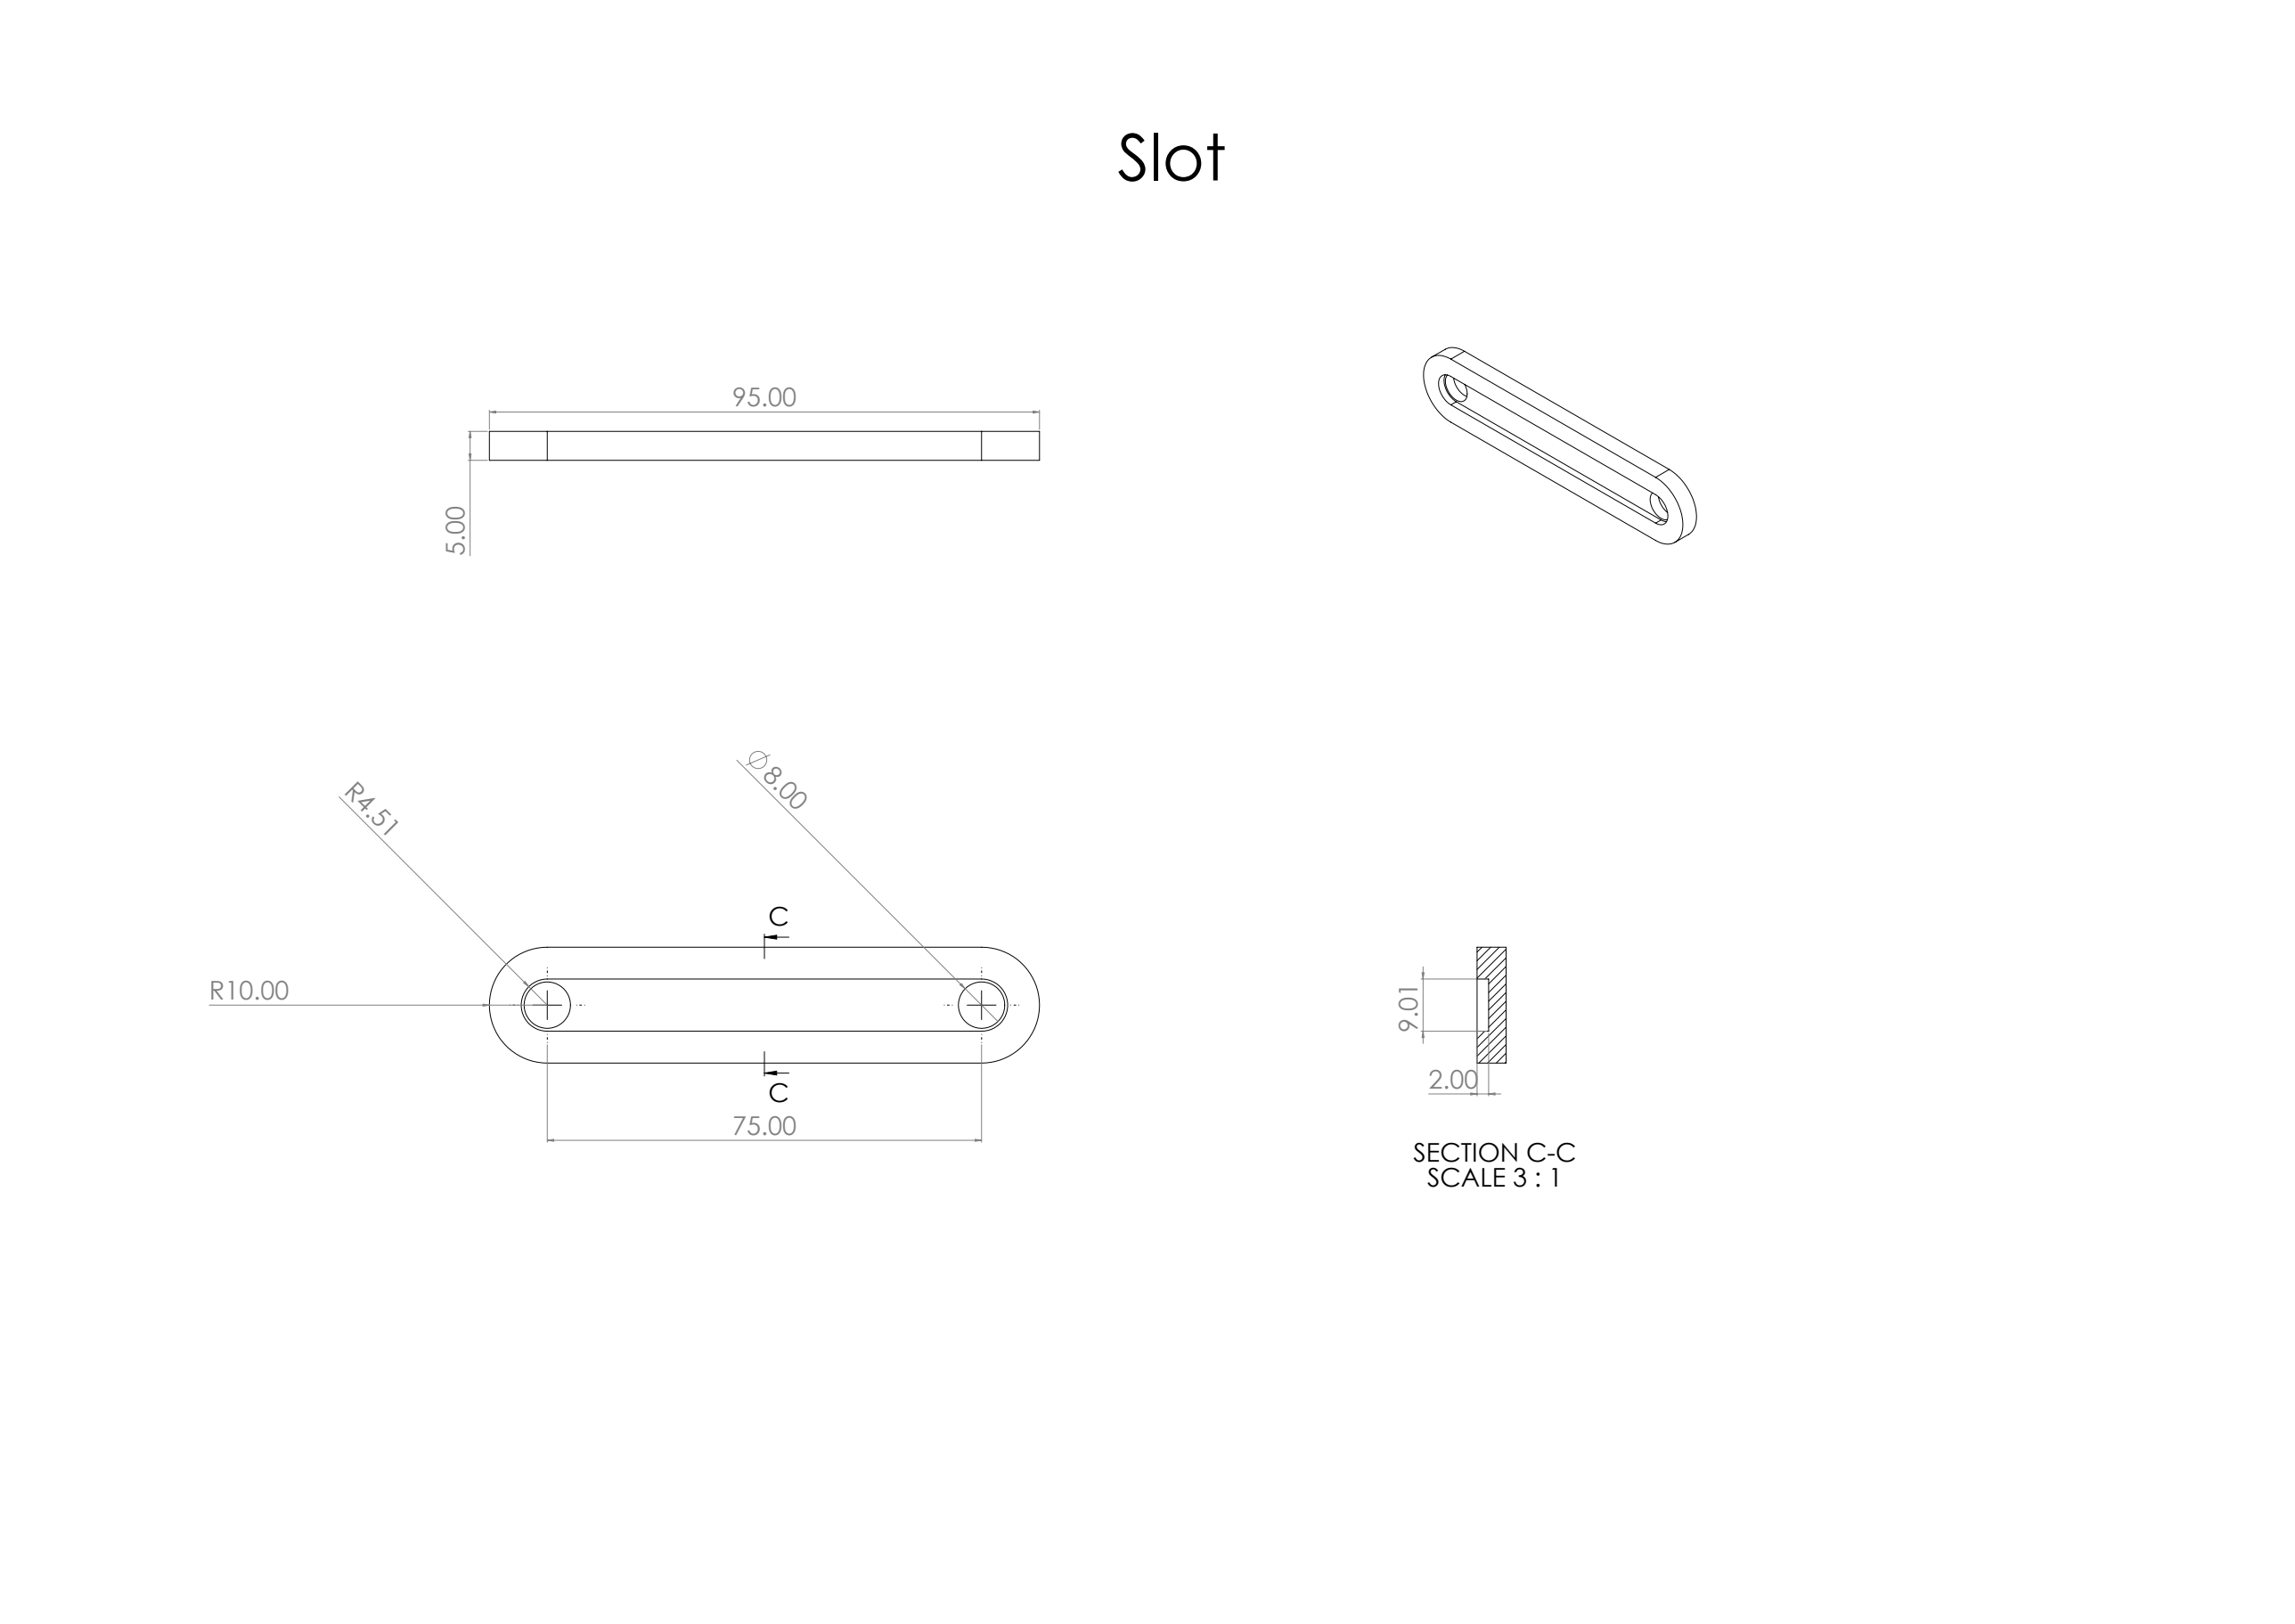
ISO-10303-21;
HEADER;
FILE_DESCRIPTION (('STEP AP214'),
    '1' );
FILE_NAME ('Slot.step',
    '2026-10-24T21:31:31',
    ( '' ),
    ( '' ),
    'SwSTEP 2.0',
    'SolidWorks 2025',
    '' );
FILE_SCHEMA (( 'AUTOMOTIVE_DESIGN' ));
ENDSEC;

DATA;
#16=CARTESIAN_POINT ( 'NONE',  ( 58.00000000000000711, -2.249290599286311032, 36.00000000000012079 ) ) ;
#145=ORIENTED_EDGE ( 'NONE', *, *, #4688, .T. ) ;
#181=CIRCLE ( 'NONE', #13427, 4.505436745857433145 ) ;
#184=ORIENTED_EDGE ( 'NONE', *, *, #4181, .F. ) ;
#194=CARTESIAN_POINT ( 'NONE',  ( -16.99999999999998579, -2.249290599286303927, 33.00000000000012790 ) ) ;
#251=VERTEX_POINT ( 'NONE', #11733 ) ;
#262=ADVANCED_FACE ( 'NONE', ( #2849 ), #1628, .F. ) ;
#272=FACE_OUTER_BOUND ( 'NONE', #12686, .T. ) ;
#287=CIRCLE ( 'NONE', #2244, 4.000000000000000000 ) ;
#323=CARTESIAN_POINT ( 'NONE',  ( -16.99999999999998579, -2.249290599286303927, 38.00000000000012079 ) ) ;
#328=CARTESIAN_POINT ( 'NONE',  ( 62.50543674585744469, -2.249290599286311032, 36.00000000000012079 ) ) ;
#339=EDGE_CURVE ( 'NONE', #4676, #369, #5590, .T. ) ;
#357=ORIENTED_EDGE ( 'NONE', *, *, #11069, .T. ) ;
#369=VERTEX_POINT ( 'NONE', #6019 ) ;
#394=DIRECTION ( 'NONE',  ( 1.000000000000000000, -9.251858538542971581E-17, 0.000000000000000000 ) ) ;
#405=CARTESIAN_POINT ( 'NONE',  ( -16.99999999999998579, -12.24929059928630437, 38.00000000000012079 ) ) ;
#428=DIRECTION ( 'NONE',  ( 0.000000000000000000, 0.000000000000000000, 1.000000000000000000 ) ) ;
#442=DIRECTION ( 'NONE',  ( 0.000000000000000000, 0.000000000000000000, 1.000000000000000000 ) ) ;
#472=LINE ( 'NONE', #13474, #12021 ) ;
#510=DIRECTION ( 'NONE',  ( 1.000000000000000000, 0.000000000000000000, 0.000000000000000000 ) ) ;
#513=VECTOR ( 'NONE', #15204, 1000.000000000000000 ) ;
#530=AXIS2_PLACEMENT_3D ( 'NONE', #3937, #5033, #8635 ) ;
#543=CARTESIAN_POINT ( 'NONE',  ( -16.99999999999998579, -2.249290599286303927, 38.00000000000012079 ) ) ;
#557=CARTESIAN_POINT ( 'NONE',  ( -16.99999999999998579, 2.256146146571129218, 38.00000000000012079 ) ) ;
#771=CARTESIAN_POINT ( 'NONE',  ( -20.99999999999998579, -2.249290599286303927, 38.00000000000012079 ) ) ;
#810=LINE ( 'NONE', #13901, #15019 ) ;
#898=DIRECTION ( 'NONE',  ( 1.000000000000000000, 0.000000000000000000, 0.000000000000000000 ) ) ;
#902=EDGE_CURVE ( 'NONE', #251, #11798, #9174, .T. ) ;
#905=PRODUCT_DEFINITION ( 'UNKNOWN', '', #1171, #3354 ) ;
#907=CARTESIAN_POINT ( 'NONE',  ( -26.99999999999998934, -2.249290599286303927, 38.00000000000012079 ) ) ;
#963=CARTESIAN_POINT ( 'NONE',  ( 62.00000000000001421, -2.249290599286310588, 33.00000000000012790 ) ) ;
#966=LINE ( 'NONE', #2988, #12194 ) ;
#976=ORIENTED_EDGE ( 'NONE', *, *, #9709, .T. ) ;
#1001=DIRECTION ( 'NONE',  ( 1.000000000000000000, 0.000000000000000000, 0.000000000000000000 ) ) ;
#1011=CARTESIAN_POINT ( 'NONE',  ( -12.99999999999998757, -2.249290599286303483, 36.00000000000012079 ) ) ;
#1066=ORIENTED_EDGE ( 'NONE', *, *, #11069, .F. ) ;
#1085=DIRECTION ( 'NONE',  ( -0.000000000000000000, -0.000000000000000000, -1.000000000000000000 ) ) ;
#1098=FACE_OUTER_BOUND ( 'NONE', #13950, .T. ) ;
#1114=CARTESIAN_POINT ( 'NONE',  ( -16.99999999999998579, -2.249290599286303927, 36.00000000000012079 ) ) ;
#1139=EDGE_CURVE ( 'NONE', #4676, #7142, #8068, .T. ) ;
#1149=ORIENTED_EDGE ( 'NONE', *, *, #11411, .F. ) ;
#1171=PRODUCT_DEFINITION_FORMATION_WITH_SPECIFIED_SOURCE ( 'ANY', '', #1909, .NOT_KNOWN. ) ;
#1196=DIRECTION ( 'NONE',  ( -0.000000000000000000, -0.000000000000000000, 1.000000000000000000 ) ) ;
#1206=ORIENTED_EDGE ( 'NONE', *, *, #9236, .T. ) ;
#1226=EDGE_CURVE ( 'NONE', #5867, #10383, #2818, .T. ) ;
#1241=EDGE_LOOP ( 'NONE', ( #9052, #8384, #14542, #4784 ) ) ;
#1272=VECTOR ( 'NONE', #1085, 1000.000000000000000 ) ;
#1276=AXIS2_PLACEMENT_3D ( 'NONE', #9205, #12823, #13888 ) ;
#1299=VECTOR ( 'NONE', #2746, 1000.000000000000000 ) ;
#1360=CYLINDRICAL_SURFACE ( 'NONE', #11358, 10.00000000000000178 ) ;
#1372=ORIENTED_EDGE ( 'NONE', *, *, #3914, .F. ) ;
#1415=AXIS2_PLACEMENT_3D ( 'NONE', #1771, #6471, #12394 ) ;
#1418=CARTESIAN_POINT ( 'NONE',  ( -16.99999999999998579, -6.754727345143736628, 36.00000000000012079 ) ) ;
#1429=EDGE_LOOP ( 'NONE', ( #13416, #7963, #11470, #145 ) ) ;
#1432=ADVANCED_FACE ( 'NONE', ( #12427 ), #1879, .F. ) ;
#1435=ORIENTED_EDGE ( 'NONE', *, *, #5988, .T. ) ;
#1499=DIRECTION ( 'NONE',  ( 0.000000000000000000, 0.000000000000000000, 1.000000000000000000 ) ) ;
#1548=ADVANCED_FACE ( 'NONE', ( #8125 ), #12828, .F. ) ;
#1573=AXIS2_PLACEMENT_3D ( 'NONE', #13753, #7834, #7985 ) ;
#1575=CARTESIAN_POINT ( 'NONE',  ( 58.00000000000000711, -12.24929059928630970, 33.00000000000012790 ) ) ;
#1602=ORIENTED_EDGE ( 'NONE', *, *, #13204, .F. ) ;
#1609=EDGE_LOOP ( 'NONE', ( #11446, #15210 ) ) ;
#1611=EDGE_CURVE ( 'NONE', #11349, #2219, #7955, .T. ) ;
#1628=CYLINDRICAL_SURFACE ( 'NONE', #13220, 4.505436745857433145 ) ;
#1673=DIRECTION ( 'NONE',  ( 1.000000000000000000, 0.000000000000000000, -0.000000000000000000 ) ) ;
#1699=CARTESIAN_POINT ( 'NONE',  ( 58.00000000000000711, -2.249290599286311032, 36.00000000000012079 ) ) ;
#1700=ADVANCED_BREP_SHAPE_REPRESENTATION ( '', ( #9466, #6315 ), #11962 ) ;
#1717=LINE ( 'NONE', #8951, #3460 ) ;
#1771=CARTESIAN_POINT ( 'NONE',  ( 58.00000000000000711, -2.249290599286311032, 36.00000000000012079 ) ) ;
#1776=DIRECTION ( 'NONE',  ( 0.000000000000000000, 0.000000000000000000, 1.000000000000000000 ) ) ;
#1804=FACE_BOUND ( 'NONE', #3358, .T. ) ;
#1835=DIRECTION ( 'NONE',  ( -0.000000000000000000, -0.000000000000000000, -1.000000000000000000 ) ) ;
#1842=FACE_OUTER_BOUND ( 'NONE', #5321, .T. ) ;
#1845=CARTESIAN_POINT ( 'NONE',  ( 58.00000000000000711, 2.256146146571122113, 38.00000000000012079 ) ) ;
#1853=( NAMED_UNIT ( * ) PLANE_ANGLE_UNIT ( ) SI_UNIT ( $, .RADIAN. ) );
#1879=PLANE ( 'NONE',  #6472 ) ;
#1890=DIRECTION ( 'NONE',  ( 0.000000000000000000, 0.000000000000000000, 1.000000000000000000 ) ) ;
#1898=AXIS2_PLACEMENT_3D ( 'NONE', #12311, #6466, #14548 ) ;
#1904=AXIS2_PLACEMENT_3D ( 'NONE', #3072, #1835, #7844 ) ;
#1906=FACE_OUTER_BOUND ( 'NONE', #7243, .T. ) ;
#1909=PRODUCT ( 'Slot', 'Slot', '', ( #13321 ) ) ;
#1955=FACE_OUTER_BOUND ( 'NONE', #5403, .T. ) ;
#1975=CARTESIAN_POINT ( 'NONE',  ( -16.99999999999998579, -2.249290599286303927, 36.00000000000012079 ) ) ;
#2020=VECTOR ( 'NONE', #2381, 1000.000000000000000 ) ;
#2025=PLANE ( 'NONE',  #9342 ) ;
#2033=AXIS2_PLACEMENT_3D ( 'NONE', #3160, #1776, #10090 ) ;
#2040=CYLINDRICAL_SURFACE ( 'NONE', #3467, 10.00000000000000178 ) ;
#2068=LINE ( 'NONE', #4686, #10105 ) ;
#2132=CIRCLE ( 'NONE', #8294, 4.000000000000000000 ) ;
#2198=DIRECTION ( 'NONE',  ( 1.000000000000000000, 0.000000000000000000, 0.000000000000000000 ) ) ;
#2219=VERTEX_POINT ( 'NONE', #1845 ) ;
#2240=ORIENTED_EDGE ( 'NONE', *, *, #1611, .F. ) ;
#2244=AXIS2_PLACEMENT_3D ( 'NONE', #3620, #8329, #6091 ) ;
#2296=DIRECTION ( 'NONE',  ( 1.000000000000000000, 0.000000000000000000, 0.000000000000000000 ) ) ;
#2306=AXIS2_PLACEMENT_3D ( 'NONE', #4421, #12665, #2198 ) ;
#2323=EDGE_CURVE ( 'NONE', #369, #4676, #10110, .T. ) ;
#2381=DIRECTION ( 'NONE',  ( -1.000000000000000000, 2.312964634635742895E-17, -0.000000000000000000 ) ) ;
#2399=FACE_OUTER_BOUND ( 'NONE', #1241, .T. ) ;
#2462=LINE ( 'NONE', #7151, #2020 ) ;
#2521=EDGE_CURVE ( 'NONE', #4675, #11128, #287, .T. ) ;
#2523=AXIS2_PLACEMENT_3D ( 'NONE', #323, #6178, #9568 ) ;
#2530=EDGE_LOOP ( 'NONE', ( #5795, #11208, #11838, #4778 ) ) ;
#2604=ORIENTED_EDGE ( 'NONE', *, *, #9709, .F. ) ;
#2676=ORIENTED_EDGE ( 'NONE', *, *, #3302, .F. ) ;
#2701=AXIS2_PLACEMENT_3D ( 'NONE', #12923, #7426, #2296 ) ;
#2709=ADVANCED_FACE ( 'NONE', ( #1955 ), #2040, .T. ) ;
#2737=ORIENTED_EDGE ( 'NONE', *, *, #5225, .T. ) ;
#2746=DIRECTION ( 'NONE',  ( -1.000000000000000000, 2.312964634635742895E-17, -0.000000000000000000 ) ) ;
#2749=CARTESIAN_POINT ( 'NONE',  ( 58.00000000000000711, -2.249290599286311032, 36.00000000000012079 ) ) ;
#2762=AXIS2_PLACEMENT_3D ( 'NONE', #16, #11860, #1001 ) ;
#2789=DIRECTION ( 'NONE',  ( -0.000000000000000000, -0.000000000000000000, -1.000000000000000000 ) ) ;
#2818=LINE ( 'NONE', #10981, #1299 ) ;
#2829=CARTESIAN_POINT ( 'NONE',  ( 58.00000000000000711, 2.256146146571122113, 36.00000000000012079 ) ) ;
#2838=ORIENTED_EDGE ( 'NONE', *, *, #13570, .T. ) ;
#2849=FACE_OUTER_BOUND ( 'NONE', #9522, .T. ) ;
#2877=CARTESIAN_POINT ( 'NONE',  ( 58.00000000000000711, 7.750709400713694741, 33.00000000000012790 ) ) ;
#2924=EDGE_CURVE ( 'NONE', #10383, #8896, #5822, .T. ) ;
#2931=CARTESIAN_POINT ( 'NONE',  ( -16.99999999999998579, 2.256146146571129218, 36.00000000000012079 ) ) ;
#2939=CARTESIAN_POINT ( 'NONE',  ( 54.00000000000000711, -2.249290599286311032, 33.00000000000012790 ) ) ;
#2968=EDGE_CURVE ( 'NONE', #6172, #4927, #4433, .T. ) ;
#2976=CARTESIAN_POINT ( 'NONE',  ( -16.99999999999998579, -2.249290599286303927, 38.00000000000012079 ) ) ;
#2980=VECTOR ( 'NONE', #14639, 1000.000000000000000 ) ;
#2988=CARTESIAN_POINT ( 'NONE',  ( 58.00000000000000711, -6.754727345143743733, 36.00000000000012079 ) ) ;
#2991=AXIS2_PLACEMENT_3D ( 'NONE', #10271, #4410, #5656 ) ;
#3024=ORIENTED_EDGE ( 'NONE', *, *, #8643, .T. ) ;
#3060=CARTESIAN_POINT ( 'NONE',  ( 58.00000000000000711, -2.249290599286311032, 38.00000000000012079 ) ) ;
#3072=CARTESIAN_POINT ( 'NONE',  ( -16.99999999999998579, -2.249290599286303927, 38.00000000000012079 ) ) ;
#3114=SHAPE_REPRESENTATION ( 'Slot', ( #6315 ), #11962 ) ;
#3124=ORIENTED_EDGE ( 'NONE', *, *, #3628, .F. ) ;
#3160=CARTESIAN_POINT ( 'NONE',  ( 58.00000000000000711, -2.249290599286311032, 33.00000000000012790 ) ) ;
#3197=AXIS2_PLACEMENT_3D ( 'NONE', #11203, #13594, #5213 ) ;
#3206=DIRECTION ( 'NONE',  ( 1.000000000000000000, 0.000000000000000000, 0.000000000000000000 ) ) ;
#3220=APPLICATION_CONTEXT ( 'automotive_design' ) ;
#3302=EDGE_CURVE ( 'NONE', #369, #13514, #472, .T. ) ;
#3310=EDGE_CURVE ( 'NONE', #5867, #13804, #7330, .T. ) ;
#3329=CARTESIAN_POINT ( 'NONE',  ( 58.00000000000000711, 2.256146146571122113, 36.00000000000012079 ) ) ;
#3333=VERTEX_POINT ( 'NONE', #10952 ) ;
#3354=PRODUCT_DEFINITION_CONTEXT ( 'detailed design', #8324, 'design' ) ;
#3358=EDGE_LOOP ( 'NONE', ( #10086, #3124 ) ) ;
#3416=DIRECTION ( 'NONE',  ( 1.000000000000000000, -2.312964634635742895E-17, 0.000000000000000000 ) ) ;
#3451=EDGE_LOOP ( 'NONE', ( #2676, #5349, #13902, #11604 ) ) ;
#3460=VECTOR ( 'NONE', #13640, 1000.000000000000000 ) ;
#3467=AXIS2_PLACEMENT_3D ( 'NONE', #7974, #4263, #13660 ) ;
#3516=DIRECTION ( 'NONE',  ( 1.000000000000000000, 0.000000000000000000, 0.000000000000000000 ) ) ;
#3535=ORIENTED_EDGE ( 'NONE', *, *, #14400, .T. ) ;
#3583=ADVANCED_FACE ( 'NONE', ( #10554 ), #7862, .F. ) ;
#3620=CARTESIAN_POINT ( 'NONE',  ( -16.99999999999998579, -2.249290599286303927, 33.00000000000012790 ) ) ;
#3628=EDGE_CURVE ( 'NONE', #11798, #251, #12783, .T. ) ;
#3732=EDGE_LOOP ( 'NONE', ( #9194, #12086, #1206, #5379, #12814 ) ) ;
#3799=EDGE_CURVE ( 'NONE', #13514, #7142, #9341, .T. ) ;
#3900=ORIENTED_EDGE ( 'NONE', *, *, #6796, .F. ) ;
#3914=EDGE_CURVE ( 'NONE', #13135, #5290, #9962, .T. ) ;
#3930=DIRECTION ( 'NONE',  ( -1.000000000000000000, 9.251858538542971581E-17, 0.000000000000000000 ) ) ;
#3937=CARTESIAN_POINT ( 'NONE',  ( -16.99999999999998579, -2.249290599286303927, 38.00000000000012079 ) ) ;
#3949=ORIENTED_EDGE ( 'NONE', *, *, #3914, .T. ) ;
#3965=CIRCLE ( 'NONE', #530, 10.00000000000000000 ) ;
#4005=DIRECTION ( 'NONE',  ( -0.000000000000000000, -0.000000000000000000, -1.000000000000000000 ) ) ;
#4044=CYLINDRICAL_SURFACE ( 'NONE', #3197, 10.00000000000000178 ) ;
#4082=CARTESIAN_POINT ( 'NONE',  ( 0.000000000000000000, 0.000000000000000000, 0.000000000000000000 ) ) ;
#4105=FACE_BOUND ( 'NONE', #10933, .T. ) ;
#4135=DIRECTION ( 'NONE',  ( 0.000000000000000000, 0.000000000000000000, 1.000000000000000000 ) ) ;
#4175=FACE_BOUND ( 'NONE', #1609, .T. ) ;
#4181=EDGE_CURVE ( 'NONE', #4272, #13804, #6672, .T. ) ;
#4189=PLANE ( 'NONE',  #8535 ) ;
#4223=DIRECTION ( 'NONE',  ( 9.251858538542971581E-17, 1.000000000000000000, 0.000000000000000000 ) ) ;
#4263=DIRECTION ( 'NONE',  ( -0.000000000000000000, -0.000000000000000000, -1.000000000000000000 ) ) ;
#4272=VERTEX_POINT ( 'NONE', #1575 ) ;
#4288=CYLINDRICAL_SURFACE ( 'NONE', #1904, 4.000000000000000000 ) ;
#4314=ORIENTED_EDGE ( 'NONE', *, *, #7498, .T. ) ;
#4317=ADVANCED_FACE ( 'NONE', ( #272 ), #11955, .F. ) ;
#4357=LINE ( 'NONE', #11275, #11956 ) ;
#4410=DIRECTION ( 'NONE',  ( 0.000000000000000000, 0.000000000000000000, 1.000000000000000000 ) ) ;
#4421=CARTESIAN_POINT ( 'NONE',  ( -16.99999999999998579, -2.249290599286303927, 36.00000000000012079 ) ) ;
#4433=CIRCLE ( 'NONE', #12304, 4.505436745857433145 ) ;
#4512=VERTEX_POINT ( 'NONE', #14010 ) ;
#4525=DIRECTION ( 'NONE',  ( -0.000000000000000000, -0.000000000000000000, -1.000000000000000000 ) ) ;
#4563=CARTESIAN_POINT ( 'NONE',  ( -16.99999999999998579, -12.24929059928630437, 38.00000000000012079 ) ) ;
#4656=VECTOR ( 'NONE', #2789, 1000.000000000000000 ) ;
#4666=AXIS2_PLACEMENT_3D ( 'NONE', #15168, #10475, #8009 ) ;
#4675=VERTEX_POINT ( 'NONE', #11547 ) ;
#4676=VERTEX_POINT ( 'NONE', #13948 ) ;
#4686=CARTESIAN_POINT ( 'NONE',  ( 62.50543674585744469, -2.249290599286311032, 36.00000000000012079 ) ) ;
#4688=EDGE_CURVE ( 'NONE', #14170, #9032, #11314, .T. ) ;
#4751=DIRECTION ( 'NONE',  ( 1.000000000000000000, 0.000000000000000000, 0.000000000000000000 ) ) ;
#4778=ORIENTED_EDGE ( 'NONE', *, *, #9015, .T. ) ;
#4784=ORIENTED_EDGE ( 'NONE', *, *, #11562, .T. ) ;
#4893=EDGE_LOOP ( 'NONE', ( #1372, #8177, #14989, #976 ) ) ;
#4898=DIRECTION ( 'NONE',  ( 0.000000000000000000, 0.000000000000000000, 1.000000000000000000 ) ) ;
#4916=CARTESIAN_POINT ( 'NONE',  ( -16.99999999999998579, 2.256146146571129218, 36.00000000000012079 ) ) ;
#4922=ORIENTED_EDGE ( 'NONE', *, *, #13204, .T. ) ;
#4923=EDGE_CURVE ( 'NONE', #4512, #6172, #14408, .T. ) ;
#4927=VERTEX_POINT ( 'NONE', #328 ) ;
#4962=DIRECTION ( 'NONE',  ( 1.000000000000000000, -9.251858538542971581E-17, 0.000000000000000000 ) ) ;
#5033=DIRECTION ( 'NONE',  ( 0.000000000000000000, 0.000000000000000000, 1.000000000000000000 ) ) ;
#5093=LINE ( 'NONE', #13389, #8004 ) ;
#5097=DIRECTION ( 'NONE',  ( 1.000000000000000000, 0.000000000000000000, 0.000000000000000000 ) ) ;
#5163=CARTESIAN_POINT ( 'NONE',  ( 58.00000000000000711, -6.754727345143743733, 38.00000000000012079 ) ) ;
#5182=CIRCLE ( 'NONE', #11818, 4.505436745857433145 ) ;
#5213=DIRECTION ( 'NONE',  ( -1.000000000000000000, 0.000000000000000000, 0.000000000000000000 ) ) ;
#5225=EDGE_CURVE ( 'NONE', #13804, #8896, #2462, .T. ) ;
#5242=PLANE ( 'NONE',  #8272 ) ;
#5290=VERTEX_POINT ( 'NONE', #8679 ) ;
#5321=EDGE_LOOP ( 'NONE', ( #10858, #9774, #1602, #5841 ) ) ;
#5349=ORIENTED_EDGE ( 'NONE', *, *, #2323, .T. ) ;
#5362=DIRECTION ( 'NONE',  ( 0.000000000000000000, 0.000000000000000000, 1.000000000000000000 ) ) ;
#5379=ORIENTED_EDGE ( 'NONE', *, *, #8061, .T. ) ;
#5403=EDGE_LOOP ( 'NONE', ( #11144, #3949, #357, #6231 ) ) ;
#5432=DIRECTION ( 'NONE',  ( -1.000000000000000000, 6.938893903907228378E-17, 0.000000000000000000 ) ) ;
#5471=ADVANCED_FACE ( 'NONE', ( #14671 ), #10296, .F. ) ;
#5494=AXIS2_PLACEMENT_3D ( 'NONE', #1975, #4135, #898 ) ;
#5561=DIRECTION ( 'NONE',  ( -0.000000000000000000, -0.000000000000000000, -1.000000000000000000 ) ) ;
#5578=ORIENTED_EDGE ( 'NONE', *, *, #2968, .T. ) ;
#5590=CIRCLE ( 'NONE', #1415, 4.000000000000003553 ) ;
#5648=( GEOMETRIC_REPRESENTATION_CONTEXT ( 3 ) GLOBAL_UNCERTAINTY_ASSIGNED_CONTEXT ( ( #13207 ) ) GLOBAL_UNIT_ASSIGNED_CONTEXT ( ( #6778, #1853, #9097 ) ) REPRESENTATION_CONTEXT ( 'NONE', 'WORKASPACE' ) );
#5656=DIRECTION ( 'NONE',  ( 1.000000000000000000, 0.000000000000000000, -0.000000000000000000 ) ) ;
#5688=AXIS2_PLACEMENT_3D ( 'NONE', #10989, #5362, #510 ) ;
#5760=CARTESIAN_POINT ( 'NONE',  ( -16.99999999999998579, 2.256146146571129218, 38.00000000000012079 ) ) ;
#5793=ADVANCED_FACE ( 'NONE', ( #9904 ), #1360, .T. ) ;
#5795=ORIENTED_EDGE ( 'NONE', *, *, #4181, .T. ) ;
#5822=LINE ( 'NONE', #10513, #513 ) ;
#5841=ORIENTED_EDGE ( 'NONE', *, *, #1611, .T. ) ;
#5867=VERTEX_POINT ( 'NONE', #14416 ) ;
#5988=EDGE_CURVE ( 'NONE', #7142, #13514, #13836, .T. ) ;
#6019=CARTESIAN_POINT ( 'NONE',  ( 62.00000000000001421, -2.249290599286310588, 36.00000000000012079 ) ) ;
#6046=EDGE_CURVE ( 'NONE', #10383, #13135, #8439, .T. ) ;
#6062=DIRECTION ( 'NONE',  ( -0.000000000000000000, -0.000000000000000000, -1.000000000000000000 ) ) ;
#6091=DIRECTION ( 'NONE',  ( 1.000000000000000000, 0.000000000000000000, 0.000000000000000000 ) ) ;
#6172=VERTEX_POINT ( 'NONE', #9088 ) ;
#6178=DIRECTION ( 'NONE',  ( 0.000000000000000000, 0.000000000000000000, 1.000000000000000000 ) ) ;
#6231=ORIENTED_EDGE ( 'NONE', *, *, #4688, .F. ) ;
#6247=EDGE_LOOP ( 'NONE', ( #2604, #7280, #184, #8906, #1066 ) ) ;
#6255=ORIENTED_EDGE ( 'NONE', *, *, #12109, .F. ) ;
#6272=CARTESIAN_POINT ( 'NONE',  ( 58.00000000000000711, -2.249290599286311032, 36.00000000000012079 ) ) ;
#6284=CARTESIAN_POINT ( 'NONE',  ( -16.99999999999998579, -2.249290599286303927, 38.00000000000012079 ) ) ;
#6315=AXIS2_PLACEMENT_3D ( 'NONE', #4082, #8567, #11096 ) ;
#6323=FACE_OUTER_BOUND ( 'NONE', #8577, .T. ) ;
#6378=STYLED_ITEM('',(#15258),#9466);
#6417=ORIENTED_EDGE ( 'NONE', *, *, #3628, .T. ) ;
#6466=DIRECTION ( 'NONE',  ( -0.000000000000000000, -0.000000000000000000, -1.000000000000000000 ) ) ;
#6471=DIRECTION ( 'NONE',  ( 0.000000000000000000, 0.000000000000000000, 1.000000000000000000 ) ) ;
#6472=AXIS2_PLACEMENT_3D ( 'NONE', #11265, #8730, #5432 ) ;
#6530=DIRECTION ( 'NONE',  ( 0.000000000000000000, 0.000000000000000000, 1.000000000000000000 ) ) ;
#6558=CARTESIAN_POINT ( 'NONE',  ( -26.99999999999998934, -2.249290599286303927, 38.00000000000012079 ) ) ;
#6590=DIRECTION ( 'NONE',  ( 1.000000000000000000, 0.000000000000000000, 0.000000000000000000 ) ) ;
#6628=( NAMED_UNIT ( * ) SI_UNIT ( $, .STERADIAN. ) SOLID_ANGLE_UNIT ( ) );
#6642=ORIENTED_EDGE ( 'NONE', *, *, #1139, .F. ) ;
#6664=DIRECTION ( 'NONE',  ( 1.000000000000000000, -9.251858538542971581E-17, 0.000000000000000000 ) ) ;
#6672=CIRCLE ( 'NONE', #1276, 9.999999999999994671 ) ;
#6678=LINE ( 'NONE', #11217, #14459 ) ;
#6721=FACE_OUTER_BOUND ( 'NONE', #12854, .T. ) ;
#6778=( LENGTH_UNIT ( ) NAMED_UNIT ( * ) SI_UNIT ( .MILLI., .METRE. ) );
#6796=EDGE_CURVE ( 'NONE', #4927, #11349, #14209, .T. ) ;
#6845=CARTESIAN_POINT ( 'NONE',  ( 58.00000000000000711, -2.249290599286311032, 36.00000000000012079 ) ) ;
#7142=VERTEX_POINT ( 'NONE', #2939 ) ;
#7151=CARTESIAN_POINT ( 'NONE',  ( -16.99999999999998579, 7.750709400713696517, 33.00000000000012790 ) ) ;
#7152=EDGE_LOOP ( 'NONE', ( #8172, #10984, #13226, #12065, #15016 ) ) ;
#7203=UNCERTAINTY_MEASURE_WITH_UNIT (LENGTH_MEASURE( 1.000000000000000082E-05 ), #14861, 'distance_accuracy_value', 'NONE');
#7243=EDGE_LOOP ( 'NONE', ( #8133, #3535, #12945, #7847 ) ) ;
#7280=ORIENTED_EDGE ( 'NONE', *, *, #5225, .F. ) ;
#7330=LINE ( 'NONE', #9733, #4656 ) ;
#7426=DIRECTION ( 'NONE',  ( 0.000000000000000000, 0.000000000000000000, 1.000000000000000000 ) ) ;
#7445=ADVANCED_FACE ( 'NONE', ( #1906 ), #4288, .F. ) ;
#7498=EDGE_CURVE ( 'NONE', #3333, #11665, #6678, .T. ) ;
#7539=ORIENTED_EDGE ( 'NONE', *, *, #11573, .T. ) ;
#7629=DIRECTION ( 'NONE',  ( 0.000000000000000000, 0.000000000000000000, 1.000000000000000000 ) ) ;
#7633=ORIENTED_EDGE ( 'NONE', *, *, #3302, .T. ) ;
#7701=DIRECTION ( 'NONE',  ( -0.000000000000000000, -0.000000000000000000, 1.000000000000000000 ) ) ;
#7787=DIRECTION ( 'NONE',  ( -0.000000000000000000, -0.000000000000000000, -1.000000000000000000 ) ) ;
#7790=CARTESIAN_POINT ( 'NONE',  ( -16.99999999999998579, -6.754727345143736628, 38.00000000000012079 ) ) ;
#7815=ADVANCED_FACE ( 'NONE', ( #12207, #8970 ), #4189, .T. ) ;
#7829=DIRECTION ( 'NONE',  ( 1.000000000000000000, -6.938893903907228378E-17, 0.000000000000000000 ) ) ;
#7834=DIRECTION ( 'NONE',  ( -0.000000000000000000, -0.000000000000000000, -1.000000000000000000 ) ) ;
#7844=DIRECTION ( 'NONE',  ( -1.000000000000000000, 0.000000000000000000, 0.000000000000000000 ) ) ;
#7847=ORIENTED_EDGE ( 'NONE', *, *, #8643, .F. ) ;
#7862=CYLINDRICAL_SURFACE ( 'NONE', #4666, 4.000000000000003553 ) ;
#7873=VECTOR ( 'NONE', #7787, 1000.000000000000000 ) ;
#7955=LINE ( 'NONE', #3329, #13718 ) ;
#7963=ORIENTED_EDGE ( 'NONE', *, *, #9015, .F. ) ;
#7970=EDGE_CURVE ( 'NONE', #2219, #11665, #11419, .T. ) ;
#7974=CARTESIAN_POINT ( 'NONE',  ( -16.99999999999998579, -2.249290599286303927, 38.00000000000012079 ) ) ;
#7977=ORIENTED_EDGE ( 'NONE', *, *, #3799, .T. ) ;
#7985=DIRECTION ( 'NONE',  ( -1.000000000000000000, 0.000000000000000000, 0.000000000000000000 ) ) ;
#8004=VECTOR ( 'NONE', #7701, 1000.000000000000000 ) ;
#8009=DIRECTION ( 'NONE',  ( -1.000000000000000000, 0.000000000000000000, 0.000000000000000000 ) ) ;
#8061=EDGE_CURVE ( 'NONE', #13501, #5867, #13934, .T. ) ;
#8068=LINE ( 'NONE', #15077, #13110 ) ;
#8100=CARTESIAN_POINT ( 'NONE',  ( -16.99999999999998579, -12.24929059928630437, 38.00000000000012079 ) ) ;
#8102=CARTESIAN_POINT ( 'NONE',  ( 62.50543674585744469, -2.249290599286311032, 38.00000000000012079 ) ) ;
#8125=FACE_OUTER_BOUND ( 'NONE', #12385, .T. ) ;
#8133=ORIENTED_EDGE ( 'NONE', *, *, #902, .T. ) ;
#8172=ORIENTED_EDGE ( 'NONE', *, *, #14499, .F. ) ;
#8177=ORIENTED_EDGE ( 'NONE', *, *, #6046, .F. ) ;
#8240=ADVANCED_FACE ( 'NONE', ( #1098 ), #2025, .F. ) ;
#8272=AXIS2_PLACEMENT_3D ( 'NONE', #2931, #4223, #3930 ) ;
#8294=AXIS2_PLACEMENT_3D ( 'NONE', #194, #14125, #9591 ) ;
#8313=LINE ( 'NONE', #4916, #10387 ) ;
#8324=APPLICATION_CONTEXT ( 'automotive_design' ) ;
#8329=DIRECTION ( 'NONE',  ( 0.000000000000000000, 0.000000000000000000, 1.000000000000000000 ) ) ;
#8360=MECHANICAL_DESIGN_GEOMETRIC_PRESENTATION_REPRESENTATION('',(#6378),#5648);
#8384=ORIENTED_EDGE ( 'NONE', *, *, #2968, .F. ) ;
#8425=ORIENTED_EDGE ( 'NONE', *, *, #3310, .T. ) ;
#8434=VECTOR ( 'NONE', #394, 1000.000000000000000 ) ;
#8439=CIRCLE ( 'NONE', #14330, 10.00000000000000000 ) ;
#8535=AXIS2_PLACEMENT_3D ( 'NONE', #2976, #442, #1673 ) ;
#8567=DIRECTION ( 'NONE',  ( 0.000000000000000000, 0.000000000000000000, 1.000000000000000000 ) ) ;
#8577=EDGE_LOOP ( 'NONE', ( #10158, #7633, #9840, #6642 ) ) ;
#8622=CARTESIAN_POINT ( 'NONE',  ( -16.99999999999998579, -6.754727345143736628, 36.00000000000012079 ) ) ;
#8635=DIRECTION ( 'NONE',  ( 1.000000000000000000, 0.000000000000000000, 0.000000000000000000 ) ) ;
#8643=EDGE_CURVE ( 'NONE', #251, #4675, #9094, .T. ) ;
#8679=CARTESIAN_POINT ( 'NONE',  ( -26.99999999999998934, -2.249290599286303927, 33.00000000000012790 ) ) ;
#8730=DIRECTION ( 'NONE',  ( 6.938893903907228378E-17, 1.000000000000000000, -0.000000000000000000 ) ) ;
#8790=ADVANCED_FACE ( 'NONE', ( #11133 ), #4044, .T. ) ;
#8802=DIRECTION ( 'NONE',  ( 1.000000000000000000, 0.000000000000000000, -0.000000000000000000 ) ) ;
#8893=VECTOR ( 'NONE', #5561, 1000.000000000000000 ) ;
#8896=VERTEX_POINT ( 'NONE', #12762 ) ;
#8906=ORIENTED_EDGE ( 'NONE', *, *, #13485, .F. ) ;
#8951=CARTESIAN_POINT ( 'NONE',  ( 58.00000000000000711, -12.24929059928630970, 38.00000000000012079 ) ) ;
#8970=FACE_OUTER_BOUND ( 'NONE', #3732, .T. ) ;
#9015=EDGE_CURVE ( 'NONE', #13501, #4272, #1717, .T. ) ;
#9028=ORIENTED_EDGE ( 'NONE', *, *, #11573, .F. ) ;
#9032=VERTEX_POINT ( 'NONE', #14870 ) ;
#9052=ORIENTED_EDGE ( 'NONE', *, *, #13197, .F. ) ;
#9075=DIRECTION ( 'NONE',  ( 1.000000000000000000, 0.000000000000000000, 0.000000000000000000 ) ) ;
#9088=CARTESIAN_POINT ( 'NONE',  ( 58.00000000000000711, -6.754727345143743733, 36.00000000000012079 ) ) ;
#9094=LINE ( 'NONE', #771, #7873 ) ;
#9097=( NAMED_UNIT ( * ) SI_UNIT ( $, .STERADIAN. ) SOLID_ANGLE_UNIT ( ) );
#9172=DIRECTION ( 'NONE',  ( 0.000000000000000000, 0.000000000000000000, 1.000000000000000000 ) ) ;
#9174=CIRCLE ( 'NONE', #5494, 4.000000000000000000 ) ;
#9194=ORIENTED_EDGE ( 'NONE', *, *, #6046, .T. ) ;
#9203=ORIENTED_EDGE ( 'NONE', *, *, #6796, .T. ) ;
#9205=CARTESIAN_POINT ( 'NONE',  ( 58.00000000000000711, -2.249290599286307479, 33.00000000000012790 ) ) ;
#9236=EDGE_CURVE ( 'NONE', #14170, #13501, #10423, .T. ) ;
#9244=DIRECTION ( 'NONE',  ( 1.000000000000000000, 0.000000000000000000, 0.000000000000000000 ) ) ;
#9252=CIRCLE ( 'NONE', #14897, 10.00000000000000000 ) ;
#9267=AXIS2_PLACEMENT_3D ( 'NONE', #9445, #12042, #3516 ) ;
#9341=CIRCLE ( 'NONE', #2701, 4.000000000000003553 ) ;
#9342=AXIS2_PLACEMENT_3D ( 'NONE', #13961, #10268, #3416 ) ;
#9348=VERTEX_POINT ( 'NONE', #7790 ) ;
#9445=CARTESIAN_POINT ( 'NONE',  ( 58.00000000000000711, -2.249290599286307479, 38.00000000000012079 ) ) ;
#9466=MANIFOLD_SOLID_BREP ( 'Cut-Extrude3', #12982 ) ;
#9522=EDGE_LOOP ( 'NONE', ( #3900, #12354, #12636, #2240 ) ) ;
#9568=DIRECTION ( 'NONE',  ( 1.000000000000000000, 0.000000000000000000, 0.000000000000000000 ) ) ;
#9591=DIRECTION ( 'NONE',  ( 1.000000000000000000, 0.000000000000000000, 0.000000000000000000 ) ) ;
#9632=CIRCLE ( 'NONE', #5688, 4.505436745857433145 ) ;
#9660=AXIS2_PLACEMENT_3D ( 'NONE', #1418, #14359, #4962 ) ;
#9666=AXIS2_PLACEMENT_3D ( 'NONE', #13353, #428, #8802 ) ;
#9702=ORIENTED_EDGE ( 'NONE', *, *, #14499, .T. ) ;
#9709=EDGE_CURVE ( 'NONE', #8896, #5290, #9252, .T. ) ;
#9733=CARTESIAN_POINT ( 'NONE',  ( 58.00000000000000711, 7.750709400713694741, 38.00000000000012079 ) ) ;
#9774=ORIENTED_EDGE ( 'NONE', *, *, #7498, .F. ) ;
#9840=ORIENTED_EDGE ( 'NONE', *, *, #5988, .F. ) ;
#9888=DIRECTION ( 'NONE',  ( 1.000000000000000000, 0.000000000000000000, 0.000000000000000000 ) ) ;
#9904=FACE_OUTER_BOUND ( 'NONE', #4893, .T. ) ;
#9962=LINE ( 'NONE', #6558, #2980 ) ;
#10027=SHAPE_REPRESENTATION_RELATIONSHIP ( 'NONE' , 'NONE' ,  #3114, #1700 ) ;
#10086=ORIENTED_EDGE ( 'NONE', *, *, #902, .F. ) ;
#10090=DIRECTION ( 'NONE',  ( 1.000000000000000000, 0.000000000000000000, 0.000000000000000000 ) ) ;
#10105=VECTOR ( 'NONE', #10612, 1000.000000000000000 ) ;
#10110=CIRCLE ( 'NONE', #15024, 4.000000000000003553 ) ;
#10158=ORIENTED_EDGE ( 'NONE', *, *, #339, .T. ) ;
#10193=PLANE ( 'NONE',  #2991 ) ;
#10268=DIRECTION ( 'NONE',  ( -2.312964634635742895E-17, -1.000000000000000000, 0.000000000000000000 ) ) ;
#10271=CARTESIAN_POINT ( 'NONE',  ( -16.99999999999998579, -2.249290599286303927, 36.00000000000012079 ) ) ;
#10296=CYLINDRICAL_SURFACE ( 'NONE', #1573, 4.000000000000000000 ) ;
#10311=VECTOR ( 'NONE', #12729, 1000.000000000000000 ) ;
#10383=VERTEX_POINT ( 'NONE', #13045 ) ;
#10387=VECTOR ( 'NONE', #13151, 1000.000000000000000 ) ;
#10416=ORIENTED_EDGE ( 'NONE', *, *, #4923, .F. ) ;
#10423=LINE ( 'NONE', #4563, #10311 ) ;
#10439=DIRECTION ( 'NONE',  ( -1.000000000000000000, 9.251858538542971581E-17, -0.000000000000000000 ) ) ;
#10475=DIRECTION ( 'NONE',  ( -0.000000000000000000, -0.000000000000000000, -1.000000000000000000 ) ) ;
#10513=CARTESIAN_POINT ( 'NONE',  ( -16.99999999999998579, 7.750709400713696517, 38.00000000000012079 ) ) ;
#10554=FACE_OUTER_BOUND ( 'NONE', #3451, .T. ) ;
#10612=DIRECTION ( 'NONE',  ( -0.000000000000000000, -0.000000000000000000, 1.000000000000000000 ) ) ;
#10623=ORIENTED_EDGE ( 'NONE', *, *, #4923, .T. ) ;
#10753=DIRECTION ( 'NONE',  ( -1.000000000000000000, 0.000000000000000000, 0.000000000000000000 ) ) ;
#10858=ORIENTED_EDGE ( 'NONE', *, *, #7970, .T. ) ;
#10907=PLANE ( 'NONE',  #9666 ) ;
#10920=ADVANCED_FACE ( 'NONE', ( #6323 ), #14615, .F. ) ;
#10924=VERTEX_POINT ( 'NONE', #5163 ) ;
#10933=EDGE_LOOP ( 'NONE', ( #1435, #7977 ) ) ;
#10952=CARTESIAN_POINT ( 'NONE',  ( -16.99999999999998579, 2.256146146571129218, 36.00000000000012079 ) ) ;
#10981=CARTESIAN_POINT ( 'NONE',  ( -16.99999999999998579, 7.750709400713696517, 38.00000000000012079 ) ) ;
#10984=ORIENTED_EDGE ( 'NONE', *, *, #7970, .F. ) ;
#10989=CARTESIAN_POINT ( 'NONE',  ( 58.00000000000000711, -2.249290599286311032, 38.00000000000012079 ) ) ;
#11004=AXIS2_PLACEMENT_3D ( 'NONE', #2749, #11266, #11049 ) ;
#11049=DIRECTION ( 'NONE',  ( 1.000000000000000000, 0.000000000000000000, 0.000000000000000000 ) ) ;
#11051=ORIENTED_EDGE ( 'NONE', *, *, #2924, .F. ) ;
#11069=EDGE_CURVE ( 'NONE', #5290, #9032, #13419, .T. ) ;
#11096=DIRECTION ( 'NONE',  ( 1.000000000000000000, 0.000000000000000000, 0.000000000000000000 ) ) ;
#11128=VERTEX_POINT ( 'NONE', #12862 ) ;
#11133=FACE_OUTER_BOUND ( 'NONE', #2530, .T. ) ;
#11144=ORIENTED_EDGE ( 'NONE', *, *, #14180, .F. ) ;
#11186=FACE_BOUND ( 'NONE', #13532, .T. ) ;
#11200=ORIENTED_EDGE ( 'NONE', *, *, #1226, .F. ) ;
#11203=CARTESIAN_POINT ( 'NONE',  ( 58.00000000000000711, -2.249290599286307479, 38.00000000000012079 ) ) ;
#11208=ORIENTED_EDGE ( 'NONE', *, *, #3310, .F. ) ;
#11216=ORIENTED_EDGE ( 'NONE', *, *, #11389, .T. ) ;
#11217=CARTESIAN_POINT ( 'NONE',  ( -16.99999999999998579, 2.256146146571129218, 36.00000000000012079 ) ) ;
#11265=CARTESIAN_POINT ( 'NONE',  ( -16.99999999999998579, -12.24929059928630437, 38.00000000000012079 ) ) ;
#11266=DIRECTION ( 'NONE',  ( 0.000000000000000000, 0.000000000000000000, 1.000000000000000000 ) ) ;
#11275=CARTESIAN_POINT ( 'NONE',  ( -16.99999999999998579, -6.754727345143736628, 38.00000000000012079 ) ) ;
#11298=CARTESIAN_POINT ( 'NONE',  ( -16.99999999999998579, -2.249290599286303927, 33.00000000000012790 ) ) ;
#11314=LINE ( 'NONE', #8100, #8893 ) ;
#11349=VERTEX_POINT ( 'NONE', #2829 ) ;
#11358=AXIS2_PLACEMENT_3D ( 'NONE', #6284, #6062, #10753 ) ;
#11389=EDGE_CURVE ( 'NONE', #9348, #10924, #4357, .T. ) ;
#11411=EDGE_CURVE ( 'NONE', #6172, #10924, #966, .T. ) ;
#11419=LINE ( 'NONE', #5760, #11960 ) ;
#11446=ORIENTED_EDGE ( 'NONE', *, *, #339, .F. ) ;
#11470=ORIENTED_EDGE ( 'NONE', *, *, #9236, .F. ) ;
#11547=CARTESIAN_POINT ( 'NONE',  ( -20.99999999999998579, -2.249290599286303927, 33.00000000000012790 ) ) ;
#11562=EDGE_CURVE ( 'NONE', #10924, #11787, #181, .T. ) ;
#11573=EDGE_CURVE ( 'NONE', #11128, #4675, #2132, .T. ) ;
#11604=ORIENTED_EDGE ( 'NONE', *, *, #3799, .F. ) ;
#11628=LINE ( 'NONE', #14020, #1272 ) ;
#11665=VERTEX_POINT ( 'NONE', #557 ) ;
#11703=CYLINDRICAL_SURFACE ( 'NONE', #2762, 4.505436745857433145 ) ;
#11733=CARTESIAN_POINT ( 'NONE',  ( -20.99999999999998579, -2.249290599286303927, 36.00000000000012079 ) ) ;
#11787=VERTEX_POINT ( 'NONE', #8102 ) ;
#11798=VERTEX_POINT ( 'NONE', #1011 ) ;
#11818=AXIS2_PLACEMENT_3D ( 'NONE', #1114, #4898, #4751 ) ;
#11838=ORIENTED_EDGE ( 'NONE', *, *, #8061, .F. ) ;
#11860=DIRECTION ( 'NONE',  ( -0.000000000000000000, -0.000000000000000000, 1.000000000000000000 ) ) ;
#11955=PLANE ( 'NONE',  #9660 ) ;
#11956=VECTOR ( 'NONE', #6664, 1000.000000000000000 ) ;
#11960=VECTOR ( 'NONE', #10439, 1000.000000000000000 ) ;
#11962=( GEOMETRIC_REPRESENTATION_CONTEXT ( 3 ) GLOBAL_UNCERTAINTY_ASSIGNED_CONTEXT ( ( #7203 ) ) GLOBAL_UNIT_ASSIGNED_CONTEXT ( ( #14861, #12639, #6628 ) ) REPRESENTATION_CONTEXT ( 'NONE', 'WORKASPACE' ) );
#12021=VECTOR ( 'NONE', #4005, 1000.000000000000000 ) ;
#12042=DIRECTION ( 'NONE',  ( 0.000000000000000000, 0.000000000000000000, 1.000000000000000000 ) ) ;
#12065=ORIENTED_EDGE ( 'NONE', *, *, #11562, .F. ) ;
#12086=ORIENTED_EDGE ( 'NONE', *, *, #14180, .T. ) ;
#12091=ADVANCED_FACE ( 'NONE', ( #1842 ), #5242, .F. ) ;
#12109=EDGE_CURVE ( 'NONE', #4512, #9348, #5093, .T. ) ;
#12194=VECTOR ( 'NONE', #12677, 1000.000000000000000 ) ;
#12207=FACE_BOUND ( 'NONE', #7152, .T. ) ;
#12251=DIRECTION ( 'NONE',  ( 1.000000000000000000, 0.000000000000000000, 0.000000000000000000 ) ) ;
#12304=AXIS2_PLACEMENT_3D ( 'NONE', #6272, #1499, #9888 ) ;
#12311=CARTESIAN_POINT ( 'NONE',  ( 58.00000000000000711, -2.249290599286311032, 38.00000000000012079 ) ) ;
#12354=ORIENTED_EDGE ( 'NONE', *, *, #13197, .T. ) ;
#12385=EDGE_LOOP ( 'NONE', ( #9702, #6255, #12734, #4314 ) ) ;
#12394=DIRECTION ( 'NONE',  ( 1.000000000000000000, 0.000000000000000000, 0.000000000000000000 ) ) ;
#12427=FACE_OUTER_BOUND ( 'NONE', #1429, .T. ) ;
#12437=CARTESIAN_POINT ( 'NONE',  ( -16.99999999999998579, -2.249290599286303927, 33.00000000000012790 ) ) ;
#12636=ORIENTED_EDGE ( 'NONE', *, *, #13362, .T. ) ;
#12639=( NAMED_UNIT ( * ) PLANE_ANGLE_UNIT ( ) SI_UNIT ( $, .RADIAN. ) );
#12665=DIRECTION ( 'NONE',  ( -0.000000000000000000, -0.000000000000000000, 1.000000000000000000 ) ) ;
#12677=DIRECTION ( 'NONE',  ( -0.000000000000000000, -0.000000000000000000, 1.000000000000000000 ) ) ;
#12686=EDGE_LOOP ( 'NONE', ( #11216, #1149, #10416, #12742 ) ) ;
#12729=DIRECTION ( 'NONE',  ( 1.000000000000000000, -6.938893903907228378E-17, 0.000000000000000000 ) ) ;
#12734=ORIENTED_EDGE ( 'NONE', *, *, #13570, .F. ) ;
#12742=ORIENTED_EDGE ( 'NONE', *, *, #12109, .T. ) ;
#12762=CARTESIAN_POINT ( 'NONE',  ( -16.99999999999998579, 7.750709400713696517, 33.00000000000012790 ) ) ;
#12783=CIRCLE ( 'NONE', #14252, 4.000000000000000000 ) ;
#12814=ORIENTED_EDGE ( 'NONE', *, *, #1226, .T. ) ;
#12823=DIRECTION ( 'NONE',  ( 0.000000000000000000, 0.000000000000000000, 1.000000000000000000 ) ) ;
#12828=CYLINDRICAL_SURFACE ( 'NONE', #2306, 4.505436745857433145 ) ;
#12854=EDGE_LOOP ( 'NONE', ( #2838, #10623, #5578, #9203, #4922 ) ) ;
#12862=CARTESIAN_POINT ( 'NONE',  ( -12.99999999999998757, -2.249290599286303483, 33.00000000000012790 ) ) ;
#12874=CARTESIAN_POINT ( 'NONE',  ( -16.99999999999998579, -2.249290599286303927, 36.00000000000012079 ) ) ;
#12923=CARTESIAN_POINT ( 'NONE',  ( 58.00000000000000711, -2.249290599286311032, 33.00000000000012790 ) ) ;
#12945=ORIENTED_EDGE ( 'NONE', *, *, #2521, .F. ) ;
#12982=CLOSED_SHELL ( 'NONE', ( #262, #2709, #10920, #7445, #5471, #3583, #7815, #14761, #5793, #1432, #8790, #8240, #1548, #12091, #14308, #4317, #13926 ) ) ;
#13045=CARTESIAN_POINT ( 'NONE',  ( -16.99999999999998579, 7.750709400713696517, 38.00000000000012079 ) ) ;
#13110=VECTOR ( 'NONE', #4525, 1000.000000000000000 ) ;
#13135=VERTEX_POINT ( 'NONE', #907 ) ;
#13151=DIRECTION ( 'NONE',  ( -1.000000000000000000, 9.251858538542971581E-17, -0.000000000000000000 ) ) ;
#13170=ORIENTED_EDGE ( 'NONE', *, *, #14400, .F. ) ;
#13197=EDGE_CURVE ( 'NONE', #4927, #11787, #2068, .T. ) ;
#13204=EDGE_CURVE ( 'NONE', #11349, #3333, #8313, .T. ) ;
#13207=UNCERTAINTY_MEASURE_WITH_UNIT (LENGTH_MEASURE( 1.000000000000000082E-05 ), #6778, 'distance_accuracy_value', 'NONE');
#13212=FACE_OUTER_BOUND ( 'NONE', #6247, .T. ) ;
#13220=AXIS2_PLACEMENT_3D ( 'NONE', #1699, #1196, #5097 ) ;
#13226=ORIENTED_EDGE ( 'NONE', *, *, #13362, .F. ) ;
#13321=PRODUCT_CONTEXT ( 'NONE', #3220, 'mechanical' ) ;
#13353=CARTESIAN_POINT ( 'NONE',  ( -16.99999999999998579, -2.249290599286303927, 33.00000000000012790 ) ) ;
#13362=EDGE_CURVE ( 'NONE', #11787, #2219, #9632, .T. ) ;
#13389=CARTESIAN_POINT ( 'NONE',  ( -16.99999999999998579, -6.754727345143736628, 36.00000000000012079 ) ) ;
#13416=ORIENTED_EDGE ( 'NONE', *, *, #13485, .T. ) ;
#13419=CIRCLE ( 'NONE', #14894, 10.00000000000000000 ) ;
#13427=AXIS2_PLACEMENT_3D ( 'NONE', #3060, #14899, #3206 ) ;
#13474=CARTESIAN_POINT ( 'NONE',  ( 62.00000000000001421, -2.249290599286310588, 38.00000000000012079 ) ) ;
#13485=EDGE_CURVE ( 'NONE', #9032, #4272, #810, .T. ) ;
#13501=VERTEX_POINT ( 'NONE', #14893 ) ;
#13514=VERTEX_POINT ( 'NONE', #963 ) ;
#13519=EDGE_LOOP ( 'NONE', ( #13170, #6417, #3024, #9028 ) ) ;
#13531=DIRECTION ( 'NONE',  ( -0.000000000000000000, -0.000000000000000000, 1.000000000000000000 ) ) ;
#13532=EDGE_LOOP ( 'NONE', ( #14054, #7539 ) ) ;
#13570=EDGE_CURVE ( 'NONE', #3333, #4512, #5182, .T. ) ;
#13594=DIRECTION ( 'NONE',  ( -0.000000000000000000, -0.000000000000000000, -1.000000000000000000 ) ) ;
#13640=DIRECTION ( 'NONE',  ( -0.000000000000000000, -0.000000000000000000, -1.000000000000000000 ) ) ;
#13660=DIRECTION ( 'NONE',  ( -1.000000000000000000, 0.000000000000000000, 0.000000000000000000 ) ) ;
#13718=VECTOR ( 'NONE', #13792, 1000.000000000000000 ) ;
#13753=CARTESIAN_POINT ( 'NONE',  ( -16.99999999999998579, -2.249290599286303927, 38.00000000000012079 ) ) ;
#13792=DIRECTION ( 'NONE',  ( -0.000000000000000000, -0.000000000000000000, 1.000000000000000000 ) ) ;
#13804=VERTEX_POINT ( 'NONE', #2877 ) ;
#13836=CIRCLE ( 'NONE', #2033, 4.000000000000003553 ) ;
#13859=DIRECTION ( 'NONE',  ( 1.000000000000000000, 0.000000000000000000, 0.000000000000000000 ) ) ;
#13888=DIRECTION ( 'NONE',  ( 1.000000000000000000, 0.000000000000000000, 0.000000000000000000 ) ) ;
#13901=CARTESIAN_POINT ( 'NONE',  ( -16.99999999999998579, -12.24929059928630437, 33.00000000000012790 ) ) ;
#13902=ORIENTED_EDGE ( 'NONE', *, *, #1139, .T. ) ;
#13926=ADVANCED_FACE ( 'NONE', ( #1804, #4175, #6721 ), #10193, .T. ) ;
#13934=CIRCLE ( 'NONE', #9267, 9.999999999999994671 ) ;
#13948=CARTESIAN_POINT ( 'NONE',  ( 54.00000000000000711, -2.249290599286311032, 36.00000000000012079 ) ) ;
#13950=EDGE_LOOP ( 'NONE', ( #2737, #11051, #11200, #8425 ) ) ;
#13961=CARTESIAN_POINT ( 'NONE',  ( -16.99999999999998579, 7.750709400713696517, 38.00000000000012079 ) ) ;
#14010=CARTESIAN_POINT ( 'NONE',  ( -16.99999999999998579, -6.754727345143736628, 36.00000000000012079 ) ) ;
#14013=DIRECTION ( 'NONE',  ( 0.000000000000000000, 0.000000000000000000, 1.000000000000000000 ) ) ;
#14020=CARTESIAN_POINT ( 'NONE',  ( -12.99999999999998757, -2.249290599286303483, 38.00000000000012079 ) ) ;
#14054=ORIENTED_EDGE ( 'NONE', *, *, #2521, .T. ) ;
#14125=DIRECTION ( 'NONE',  ( 0.000000000000000000, 0.000000000000000000, 1.000000000000000000 ) ) ;
#14170=VERTEX_POINT ( 'NONE', #405 ) ;
#14180=EDGE_CURVE ( 'NONE', #13135, #14170, #3965, .T. ) ;
#14209=CIRCLE ( 'NONE', #11004, 4.505436745857433145 ) ;
#14252=AXIS2_PLACEMENT_3D ( 'NONE', #12874, #9172, #13859 ) ;
#14308=ADVANCED_FACE ( 'NONE', ( #2399 ), #11703, .F. ) ;
#14330=AXIS2_PLACEMENT_3D ( 'NONE', #543, #7629, #12251 ) ;
#14359=DIRECTION ( 'NONE',  ( -9.251858538542971581E-17, -1.000000000000000000, 0.000000000000000000 ) ) ;
#14400=EDGE_CURVE ( 'NONE', #11798, #11128, #11628, .T. ) ;
#14408=LINE ( 'NONE', #8622, #8434 ) ;
#14416=CARTESIAN_POINT ( 'NONE',  ( 58.00000000000000711, 7.750709400713694741, 38.00000000000012079 ) ) ;
#14459=VECTOR ( 'NONE', #13531, 1000.000000000000000 ) ;
#14479=SHAPE_DEFINITION_REPRESENTATION ( #14813, #3114 ) ;
#14499=EDGE_CURVE ( 'NONE', #11665, #9348, #14555, .T. ) ;
#14542=ORIENTED_EDGE ( 'NONE', *, *, #11411, .T. ) ;
#14548=DIRECTION ( 'NONE',  ( -1.000000000000000000, 0.000000000000000000, 0.000000000000000000 ) ) ;
#14555=CIRCLE ( 'NONE', #2523, 4.505436745857433145 ) ;
#14615=CYLINDRICAL_SURFACE ( 'NONE', #1898, 4.000000000000003553 ) ;
#14639=DIRECTION ( 'NONE',  ( -0.000000000000000000, -0.000000000000000000, -1.000000000000000000 ) ) ;
#14671=FACE_OUTER_BOUND ( 'NONE', #13519, .T. ) ;
#14761=ADVANCED_FACE ( 'NONE', ( #13212, #11186, #4105 ), #10907, .F. ) ;
#14813=PRODUCT_DEFINITION_SHAPE ( 'NONE', 'NONE',  #905 ) ;
#14861=( LENGTH_UNIT ( ) NAMED_UNIT ( * ) SI_UNIT ( .MILLI., .METRE. ) );
#14870=CARTESIAN_POINT ( 'NONE',  ( -16.99999999999998579, -12.24929059928630437, 33.00000000000012790 ) ) ;
#14893=CARTESIAN_POINT ( 'NONE',  ( 58.00000000000000711, -12.24929059928630970, 38.00000000000012079 ) ) ;
#14894=AXIS2_PLACEMENT_3D ( 'NONE', #11298, #6530, #9075 ) ;
#14897=AXIS2_PLACEMENT_3D ( 'NONE', #12437, #1890, #6590 ) ;
#14899=DIRECTION ( 'NONE',  ( 0.000000000000000000, 0.000000000000000000, 1.000000000000000000 ) ) ;
#14989=ORIENTED_EDGE ( 'NONE', *, *, #2924, .T. ) ;
#15016=ORIENTED_EDGE ( 'NONE', *, *, #11389, .F. ) ;
#15019=VECTOR ( 'NONE', #7829, 1000.000000000000000 ) ;
#15024=AXIS2_PLACEMENT_3D ( 'NONE', #6845, #14013, #9244 ) ;
#15077=CARTESIAN_POINT ( 'NONE',  ( 54.00000000000000711, -2.249290599286311032, 38.00000000000012079 ) ) ;
#15168=CARTESIAN_POINT ( 'NONE',  ( 58.00000000000000711, -2.249290599286311032, 38.00000000000012079 ) ) ;
#15204=DIRECTION ( 'NONE',  ( -0.000000000000000000, -0.000000000000000000, -1.000000000000000000 ) ) ;
#15210=ORIENTED_EDGE ( 'NONE', *, *, #2323, .F. ) ;
#15252=COLOUR_RGB('Sky Blue',0.24,0.69,0.87);
#15253=FILL_AREA_STYLE_COLOUR('',#15252);
#15254=FILL_AREA_STYLE('',(#15253));
#15255=SURFACE_STYLE_FILL_AREA(#15254);
#15256=SURFACE_SIDE_STYLE('',(#15255));
#15257=SURFACE_STYLE_USAGE(.BOTH.,#15256);
#15258=PRESENTATION_STYLE_ASSIGNMENT((#15257));
ENDSEC;
END-ISO-10303-21;
